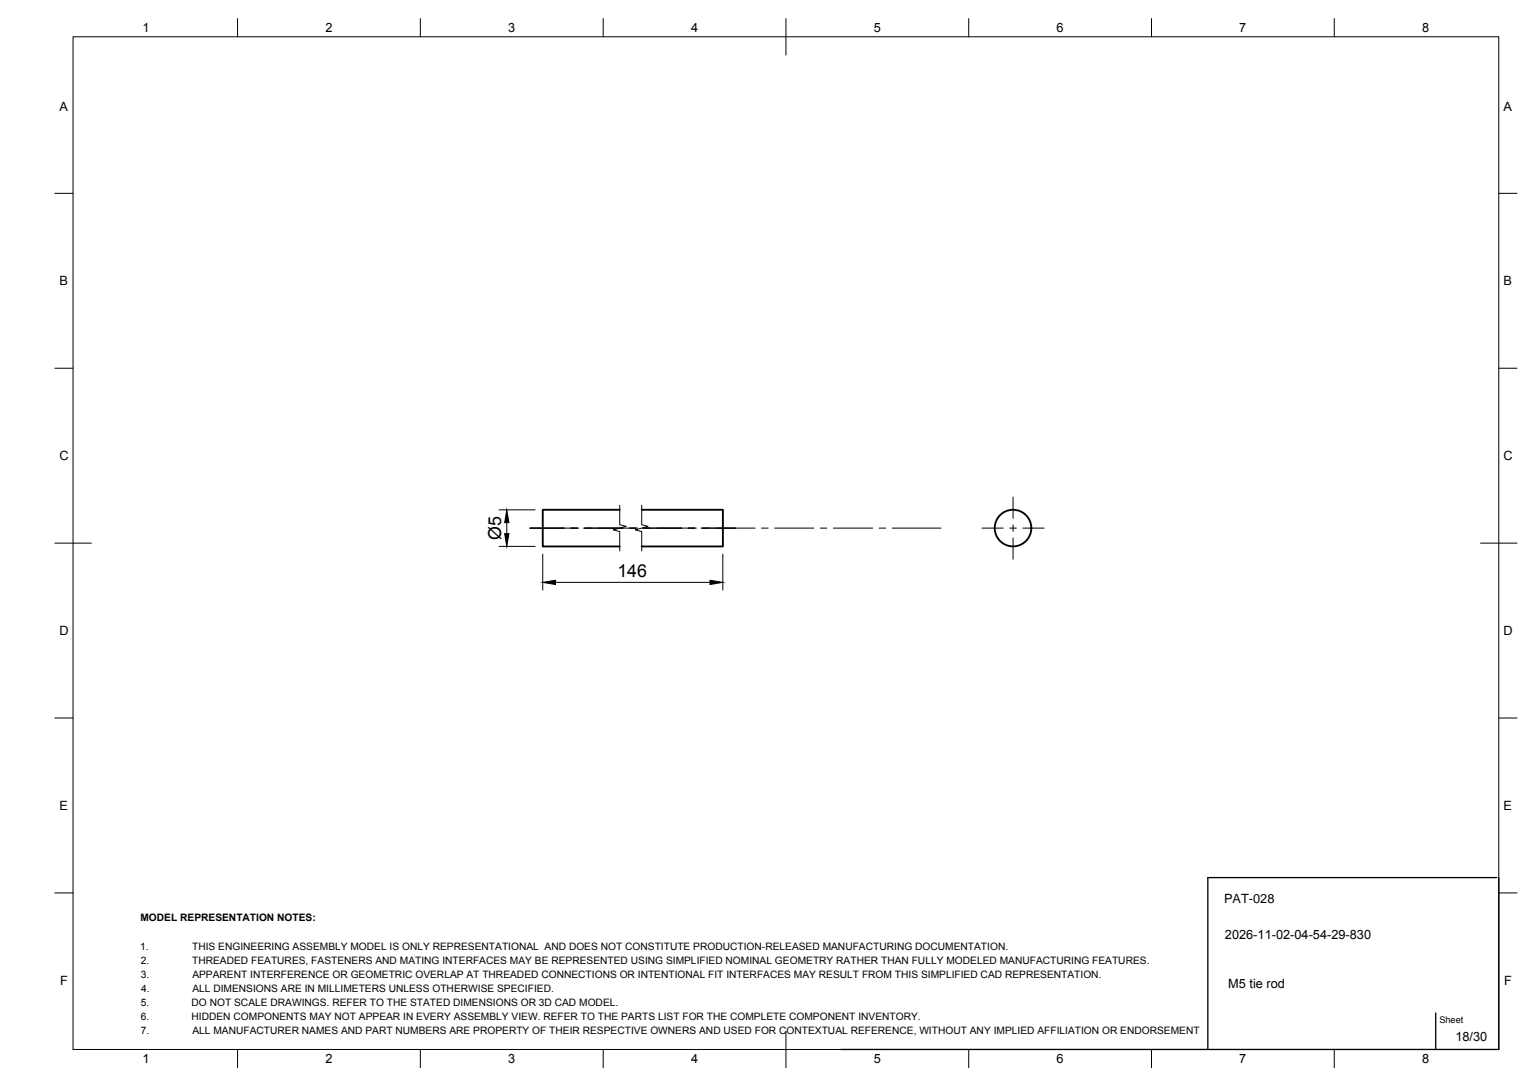
ISO-10303-21;
HEADER;
/* Generated by software containing ST-Developer
 * from STEP Tools, Inc. (www.steptools.com) 
 */

FILE_DESCRIPTION(
/* description */ ('Cylinder foot and clevis mount kit'),
/* implementation_level */ '2;1');

FILE_NAME(
/* name */ 'M5 tie rod.step',
/* time_stamp */ '2026-10-27T20:10:43-07:00',
/* author */ (''),
/* organization */ (''),
/* preprocessor_version */ 'ST-DEVELOPER v20.2',
/* originating_system */ 'Autodesk Translation Framework v15.17.0.0',
/* authorisation */ '');

FILE_SCHEMA (('AUTOMOTIVE_DESIGN { 1 0 10303 214 3 1 1 }'));
ENDSEC;

DATA;
#10=MECHANICAL_DESIGN_GEOMETRIC_PRESENTATION_REPRESENTATION('',(#354),#9102);
#298=SHAPE_REPRESENTATION_RELATIONSHIP('SRR','None',#9246,#326);
#326=ADVANCED_BREP_SHAPE_REPRESENTATION('',(#381),#9089);
#354=STYLED_ITEM('',(#9460),#381);
#381=MANIFOLD_SOLID_BREP('Body1',#4941);
#635=PLANE('',#5667);
#636=PLANE('',#5668);
#904=FACE_OUTER_BOUND('',#1288,.T.);
#905=FACE_OUTER_BOUND('',#1289,.T.);
#906=FACE_OUTER_BOUND('',#1290,.T.);
#1288=EDGE_LOOP('',(#4137,#4138,#4139,#4140));
#1289=EDGE_LOOP('',(#4141));
#1290=EDGE_LOOP('',(#4142));
#1651=LINE('',#8402,#2000);
#2000=VECTOR('',#6938,0.25);
#2264=CIRCLE('',#5665,0.25);
#2265=CIRCLE('',#5666,0.25);
#2588=VERTEX_POINT('',#8399);
#2589=VERTEX_POINT('',#8401);
#3123=EDGE_CURVE('',#2588,#2588,#2264,.T.);
#3124=EDGE_CURVE('',#2588,#2589,#1651,.T.);
#3125=EDGE_CURVE('',#2589,#2589,#2265,.T.);
#4137=ORIENTED_EDGE('',*,*,#3123,.F.);
#4138=ORIENTED_EDGE('',*,*,#3124,.T.);
#4139=ORIENTED_EDGE('',*,*,#3125,.T.);
#4140=ORIENTED_EDGE('',*,*,#3124,.F.);
#4141=ORIENTED_EDGE('',*,*,#3123,.T.);
#4142=ORIENTED_EDGE('',*,*,#3125,.F.);
#4594=CYLINDRICAL_SURFACE('',#5664,0.25);
#4827=ADVANCED_FACE('',(#904),#4594,.T.);
#4828=ADVANCED_FACE('',(#905),#635,.T.);
#4829=ADVANCED_FACE('',(#906),#636,.F.);
#4941=CLOSED_SHELL('',(#4827,#4828,#4829));
#5663=AXIS2_PLACEMENT_3D('',#8397,#6932,#6933);
#5664=AXIS2_PLACEMENT_3D('',#8398,#6934,#6935);
#5665=AXIS2_PLACEMENT_3D('',#8400,#6936,#6937);
#5666=AXIS2_PLACEMENT_3D('',#8403,#6939,#6940);
#5667=AXIS2_PLACEMENT_3D('',#8404,#6941,#6942);
#5668=AXIS2_PLACEMENT_3D('',#8405,#6943,#6944);
#6932=DIRECTION('axis',(0.,0.,1.));
#6933=DIRECTION('refdir',(1.,0.,0.));
#6934=DIRECTION('center_axis',(0.,1.,0.));
#6935=DIRECTION('ref_axis',(1.,0.,0.));
#6936=DIRECTION('center_axis',(0.,1.,0.));
#6937=DIRECTION('ref_axis',(1.,0.,0.));
#6938=DIRECTION('',(0.,-1.,0.));
#6939=DIRECTION('center_axis',(0.,1.,0.));
#6940=DIRECTION('ref_axis',(1.,0.,0.));
#6941=DIRECTION('center_axis',(0.,1.,0.));
#6942=DIRECTION('ref_axis',(1.,0.,0.));
#6943=DIRECTION('center_axis',(0.,1.,0.));
#6944=DIRECTION('ref_axis',(1.,0.,0.));
#8397=CARTESIAN_POINT('',(0.,0.,0.));
#8398=CARTESIAN_POINT('Origin',(-2.,-1.,2.5));
#8399=CARTESIAN_POINT('',(-2.25,13.6,2.5));
#8400=CARTESIAN_POINT('Origin',(-2.,13.6,2.5));
#8401=CARTESIAN_POINT('',(-2.25,-1.,2.5));
#8402=CARTESIAN_POINT('',(-2.25,-1.,2.5));
#8403=CARTESIAN_POINT('Origin',(-2.,-1.,2.5));
#8404=CARTESIAN_POINT('Origin',(-2.,13.6,2.5));
#8405=CARTESIAN_POINT('Origin',(-2.,-1.,2.5));
#9056=UNCERTAINTY_MEASURE_WITH_UNIT(LENGTH_MEASURE(0.001),#9103,
'DISTANCE_ACCURACY_VALUE',
'Maximum model space distance between geometric entities at asserted c
onnectivities');
#9069=UNCERTAINTY_MEASURE_WITH_UNIT(LENGTH_MEASURE(0.001),#9103,
'DISTANCE_ACCURACY_VALUE',
'Maximum model space distance between geometric entities at asserted c
onnectivities');
#9089=(
GEOMETRIC_REPRESENTATION_CONTEXT(3)
GLOBAL_UNCERTAINTY_ASSIGNED_CONTEXT((#9056))
GLOBAL_UNIT_ASSIGNED_CONTEXT((#9103,#9105,#9106))
REPRESENTATION_CONTEXT('','3D')
);
#9102=(
GEOMETRIC_REPRESENTATION_CONTEXT(3)
GLOBAL_UNCERTAINTY_ASSIGNED_CONTEXT((#9069))
GLOBAL_UNIT_ASSIGNED_CONTEXT((#9103,#9105,#9106))
REPRESENTATION_CONTEXT('','3D')
);
#9103=(
LENGTH_UNIT()
NAMED_UNIT(*)
SI_UNIT(.CENTI.,.METRE.)
);
#9105=(
NAMED_UNIT(*)
PLANE_ANGLE_UNIT()
SI_UNIT($,.RADIAN.)
);
#9106=(
NAMED_UNIT(*)
SI_UNIT($,.STERADIAN.)
SOLID_ANGLE_UNIT()
);
#9126=SHAPE_DEFINITION_REPRESENTATION(#9160,#9246);
#9160=PRODUCT_DEFINITION_SHAPE('',$,#9279);
#9246=SHAPE_REPRESENTATION('',(#5663),#9089);
#9259=PRODUCT_DEFINITION_CONTEXT('part definition',#9357,'design');
#9279=PRODUCT_DEFINITION('M5 tie rod','M5 tie rod',#9311,#9259);
#9311=PRODUCT_DEFINITION_FORMATION('',$,#9378);
#9357=APPLICATION_CONTEXT(
'Core Data for Automotive Mechanical Design Process');
#9358=PRODUCT_CONTEXT('part definition',#9357,'mechanical');
#9378=PRODUCT('M5 tie rod','M5 tie rod','M5 tie rod',(#9358));
#9454=COLOUR_RGB('Grey',0.48,0.52,0.57);
#9455=FILL_AREA_STYLE_COLOUR('',#9454);
#9456=FILL_AREA_STYLE('',(#9455));
#9457=SURFACE_STYLE_FILL_AREA(#9456);
#9458=SURFACE_SIDE_STYLE('',(#9457));
#9459=SURFACE_STYLE_USAGE(.BOTH.,#9458);
#9460=PRESENTATION_STYLE_ASSIGNMENT((#9459));
ENDSEC;
END-ISO-10303-21;
